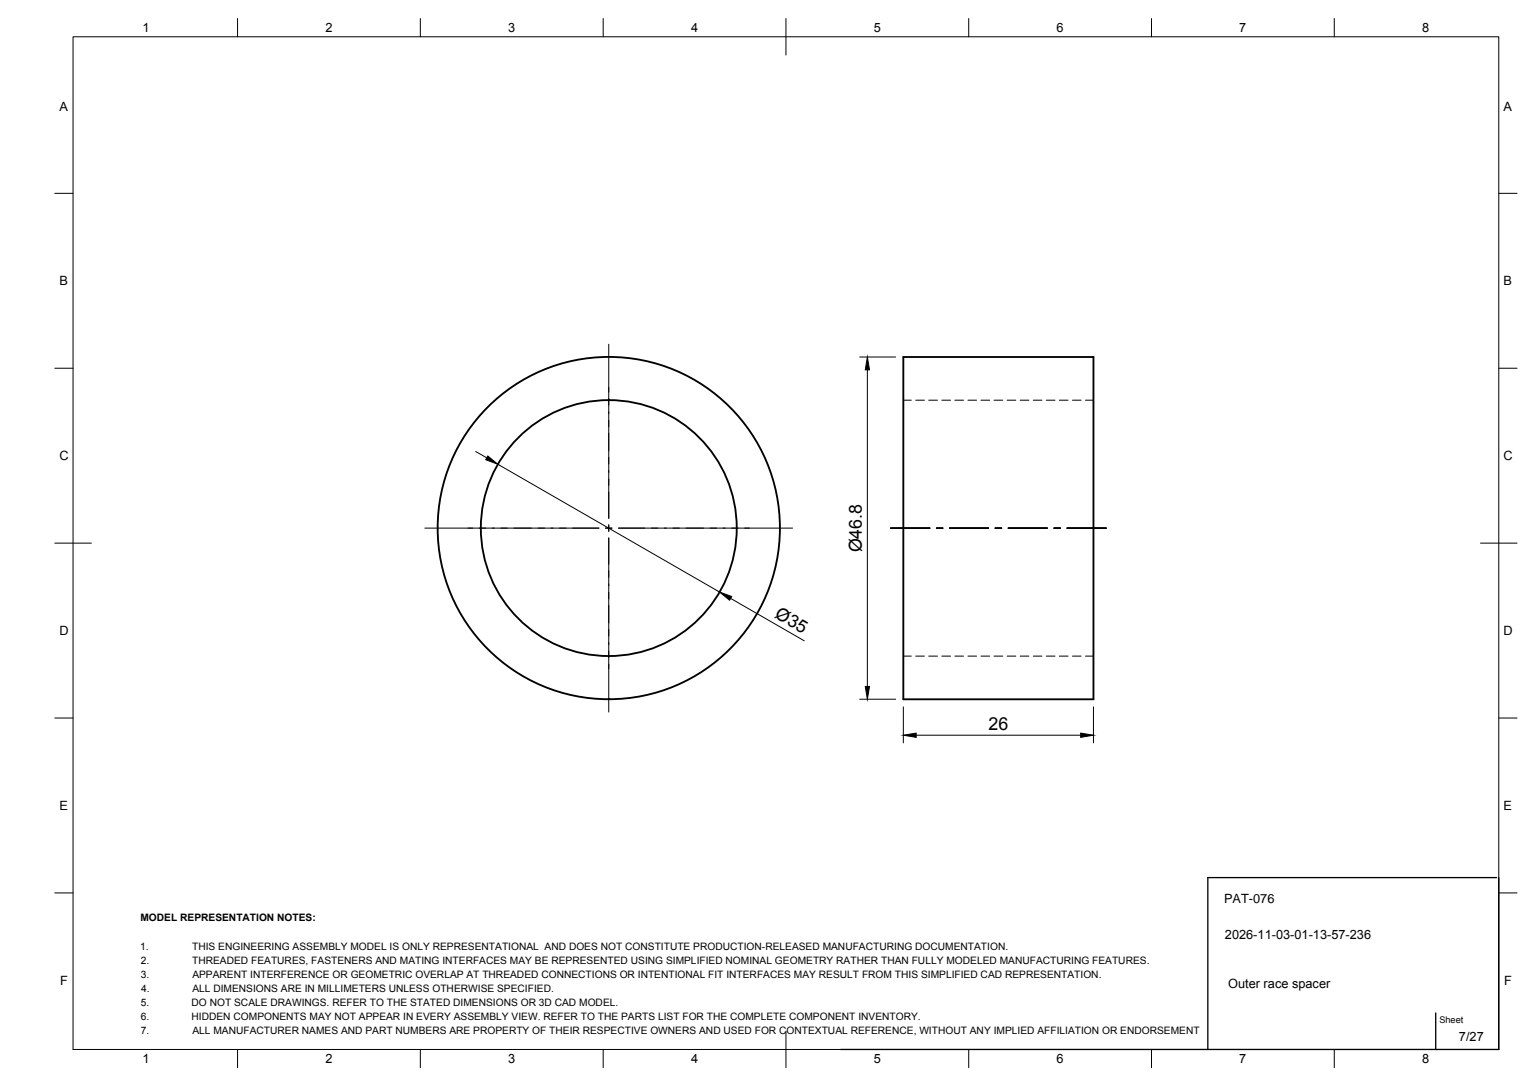
ISO-10303-21;
HEADER;
/* Generated by software containing ST-Developer
 * from STEP Tools, Inc. (www.steptools.com) 
 */

FILE_DESCRIPTION(
/* description */ ('Overhung pulley bearing cartridge'),
/* implementation_level */ '2;1');

FILE_NAME(
/* name */ 'Outer race spacer.step',
/* time_stamp */ '2026-10-28T03:22:33-07:00',
/* author */ (''),
/* organization */ (''),
/* preprocessor_version */ 'ST-DEVELOPER v20.2',
/* originating_system */ 'Autodesk Translation Framework v15.17.0.0',
/* authorisation */ '');

FILE_SCHEMA (('AUTOMOTIVE_DESIGN { 1 0 10303 214 3 1 1 }'));
ENDSEC;

DATA;
#10=MECHANICAL_DESIGN_GEOMETRIC_PRESENTATION_REPRESENTATION('',(#285),#10963);
#241=SHAPE_REPRESENTATION_RELATIONSHIP('SRR','None',#11061,#263);
#263=ADVANCED_BREP_SHAPE_REPRESENTATION('',(#315),#10941);
#285=STYLED_ITEM('',(#11253),#315);
#315=MANIFOLD_SOLID_BREP('Body1',#5652);
#369=FACE_BOUND('',#989,.T.);
#370=FACE_BOUND('',#991,.T.);
#468=PLANE('',#6032);
#469=PLANE('',#6033);
#629=FACE_OUTER_BOUND('',#986,.T.);
#630=FACE_OUTER_BOUND('',#987,.T.);
#631=FACE_OUTER_BOUND('',#988,.T.);
#632=FACE_OUTER_BOUND('',#990,.T.);
#986=EDGE_LOOP('',(#3873,#3874,#3875,#3876));
#987=EDGE_LOOP('',(#3877,#3878,#3879,#3880));
#988=EDGE_LOOP('',(#3881));
#989=EDGE_LOOP('',(#3882));
#990=EDGE_LOOP('',(#3883));
#991=EDGE_LOOP('',(#3884));
#1394=LINE('',#8799,#1736);
#1395=LINE('',#8805,#1737);
#1736=VECTOR('',#6960,1.75);
#1737=VECTOR('',#6967,2.34);
#2056=CIRCLE('',#6027,1.75);
#2057=CIRCLE('',#6028,1.75);
#2058=CIRCLE('',#6030,2.34);
#2059=CIRCLE('',#6031,2.34);
#2455=VERTEX_POINT('',#8796);
#2456=VERTEX_POINT('',#8798);
#2457=VERTEX_POINT('',#8802);
#2458=VERTEX_POINT('',#8804);
#3006=EDGE_CURVE('',#2455,#2455,#2056,.T.);
#3007=EDGE_CURVE('',#2455,#2456,#1394,.T.);
#3008=EDGE_CURVE('',#2456,#2456,#2057,.T.);
#3009=EDGE_CURVE('',#2457,#2457,#2058,.T.);
#3010=EDGE_CURVE('',#2457,#2458,#1395,.T.);
#3011=EDGE_CURVE('',#2458,#2458,#2059,.T.);
#3873=ORIENTED_EDGE('',*,*,#3006,.F.);
#3874=ORIENTED_EDGE('',*,*,#3007,.T.);
#3875=ORIENTED_EDGE('',*,*,#3008,.T.);
#3876=ORIENTED_EDGE('',*,*,#3007,.F.);
#3877=ORIENTED_EDGE('',*,*,#3009,.F.);
#3878=ORIENTED_EDGE('',*,*,#3010,.T.);
#3879=ORIENTED_EDGE('',*,*,#3011,.T.);
#3880=ORIENTED_EDGE('',*,*,#3010,.F.);
#3881=ORIENTED_EDGE('',*,*,#3009,.T.);
#3882=ORIENTED_EDGE('',*,*,#3006,.T.);
#3883=ORIENTED_EDGE('',*,*,#3011,.F.);
#3884=ORIENTED_EDGE('',*,*,#3008,.F.);
#5185=CYLINDRICAL_SURFACE('',#6026,1.75);
#5186=CYLINDRICAL_SURFACE('',#6029,2.34);
#5373=ADVANCED_FACE('',(#629),#5185,.F.);
#5374=ADVANCED_FACE('',(#630),#5186,.T.);
#5375=ADVANCED_FACE('',(#631,#369),#468,.T.);
#5376=ADVANCED_FACE('',(#632,#370),#469,.F.);
#5652=CLOSED_SHELL('',(#5373,#5374,#5375,#5376));
#6025=AXIS2_PLACEMENT_3D('',#8794,#6954,#6955);
#6026=AXIS2_PLACEMENT_3D('',#8795,#6956,#6957);
#6027=AXIS2_PLACEMENT_3D('',#8797,#6958,#6959);
#6028=AXIS2_PLACEMENT_3D('',#8800,#6961,#6962);
#6029=AXIS2_PLACEMENT_3D('',#8801,#6963,#6964);
#6030=AXIS2_PLACEMENT_3D('',#8803,#6965,#6966);
#6031=AXIS2_PLACEMENT_3D('',#8806,#6968,#6969);
#6032=AXIS2_PLACEMENT_3D('',#8807,#6970,#6971);
#6033=AXIS2_PLACEMENT_3D('',#8808,#6972,#6973);
#6954=DIRECTION('axis',(0.,0.,1.));
#6955=DIRECTION('refdir',(1.,0.,0.));
#6956=DIRECTION('center_axis',(0.,1.,0.));
#6957=DIRECTION('ref_axis',(1.,0.,0.));
#6958=DIRECTION('center_axis',(0.,-1.,0.));
#6959=DIRECTION('ref_axis',(1.,0.,0.));
#6960=DIRECTION('',(0.,-1.,0.));
#6961=DIRECTION('center_axis',(0.,-1.,0.));
#6962=DIRECTION('ref_axis',(1.,0.,0.));
#6963=DIRECTION('center_axis',(0.,1.,0.));
#6964=DIRECTION('ref_axis',(1.,0.,0.));
#6965=DIRECTION('center_axis',(0.,1.,0.));
#6966=DIRECTION('ref_axis',(1.,0.,0.));
#6967=DIRECTION('',(0.,-1.,0.));
#6968=DIRECTION('center_axis',(0.,1.,0.));
#6969=DIRECTION('ref_axis',(1.,0.,0.));
#6970=DIRECTION('center_axis',(0.,1.,0.));
#6971=DIRECTION('ref_axis',(1.,0.,0.));
#6972=DIRECTION('center_axis',(0.,1.,0.));
#6973=DIRECTION('ref_axis',(1.,0.,0.));
#8794=CARTESIAN_POINT('',(0.,0.,0.));
#8795=CARTESIAN_POINT('Origin',(0.,1.7,4.5));
#8796=CARTESIAN_POINT('',(-1.75,4.3,4.5));
#8797=CARTESIAN_POINT('Origin',(0.,4.3,4.5));
#8798=CARTESIAN_POINT('',(-1.75,1.7,4.5));
#8799=CARTESIAN_POINT('',(-1.75,1.7,4.5));
#8800=CARTESIAN_POINT('Origin',(0.,1.7,4.5));
#8801=CARTESIAN_POINT('Origin',(0.,1.7,4.5));
#8802=CARTESIAN_POINT('',(-2.34,4.3,4.5));
#8803=CARTESIAN_POINT('Origin',(0.,4.3,4.5));
#8804=CARTESIAN_POINT('',(-2.34,1.7,4.5));
#8805=CARTESIAN_POINT('',(-2.34,1.7,4.5));
#8806=CARTESIAN_POINT('Origin',(0.,1.7,4.5));
#8807=CARTESIAN_POINT('Origin',(0.,4.3,4.5));
#8808=CARTESIAN_POINT('Origin',(0.,1.7,4.5));
#10914=UNCERTAINTY_MEASURE_WITH_UNIT(LENGTH_MEASURE(0.001),#10964,
'DISTANCE_ACCURACY_VALUE',
'Maximum model space distance between geometric entities at asserted c
onnectivities');
#10936=UNCERTAINTY_MEASURE_WITH_UNIT(LENGTH_MEASURE(0.001),#10964,
'DISTANCE_ACCURACY_VALUE',
'Maximum model space distance between geometric entities at asserted c
onnectivities');
#10941=(
GEOMETRIC_REPRESENTATION_CONTEXT(3)
GLOBAL_UNCERTAINTY_ASSIGNED_CONTEXT((#10914))
GLOBAL_UNIT_ASSIGNED_CONTEXT((#10964,#10966,#10967))
REPRESENTATION_CONTEXT('','3D')
);
#10963=(
GEOMETRIC_REPRESENTATION_CONTEXT(3)
GLOBAL_UNCERTAINTY_ASSIGNED_CONTEXT((#10936))
GLOBAL_UNIT_ASSIGNED_CONTEXT((#10964,#10966,#10967))
REPRESENTATION_CONTEXT('','3D')
);
#10964=(
LENGTH_UNIT()
NAMED_UNIT(*)
SI_UNIT(.CENTI.,.METRE.)
);
#10966=(
NAMED_UNIT(*)
PLANE_ANGLE_UNIT()
SI_UNIT($,.RADIAN.)
);
#10967=(
NAMED_UNIT(*)
SI_UNIT($,.STERADIAN.)
SOLID_ANGLE_UNIT()
);
#10972=SHAPE_DEFINITION_REPRESENTATION(#10998,#11061);
#10998=PRODUCT_DEFINITION_SHAPE('',$,#11088);
#11061=SHAPE_REPRESENTATION('',(#6025),#10941);
#11083=PRODUCT_DEFINITION_CONTEXT('part definition',#11163,'design');
#11088=PRODUCT_DEFINITION('Outer race spacer','Outer race spacer',#11114,
#11083);
#11114=PRODUCT_DEFINITION_FORMATION('',$,#11169);
#11163=APPLICATION_CONTEXT(
'Core Data for Automotive Mechanical Design Process');
#11164=PRODUCT_CONTEXT('part definition',#11163,'mechanical');
#11169=PRODUCT('Outer race spacer','Outer race spacer',
'Outer race spacer',(#11164));
#11247=COLOUR_RGB('Grey',0.48,0.52,0.57);
#11248=FILL_AREA_STYLE_COLOUR('',#11247);
#11249=FILL_AREA_STYLE('',(#11248));
#11250=SURFACE_STYLE_FILL_AREA(#11249);
#11251=SURFACE_SIDE_STYLE('',(#11250));
#11252=SURFACE_STYLE_USAGE(.BOTH.,#11251);
#11253=PRESENTATION_STYLE_ASSIGNMENT((#11252));
ENDSEC;
END-ISO-10303-21;
